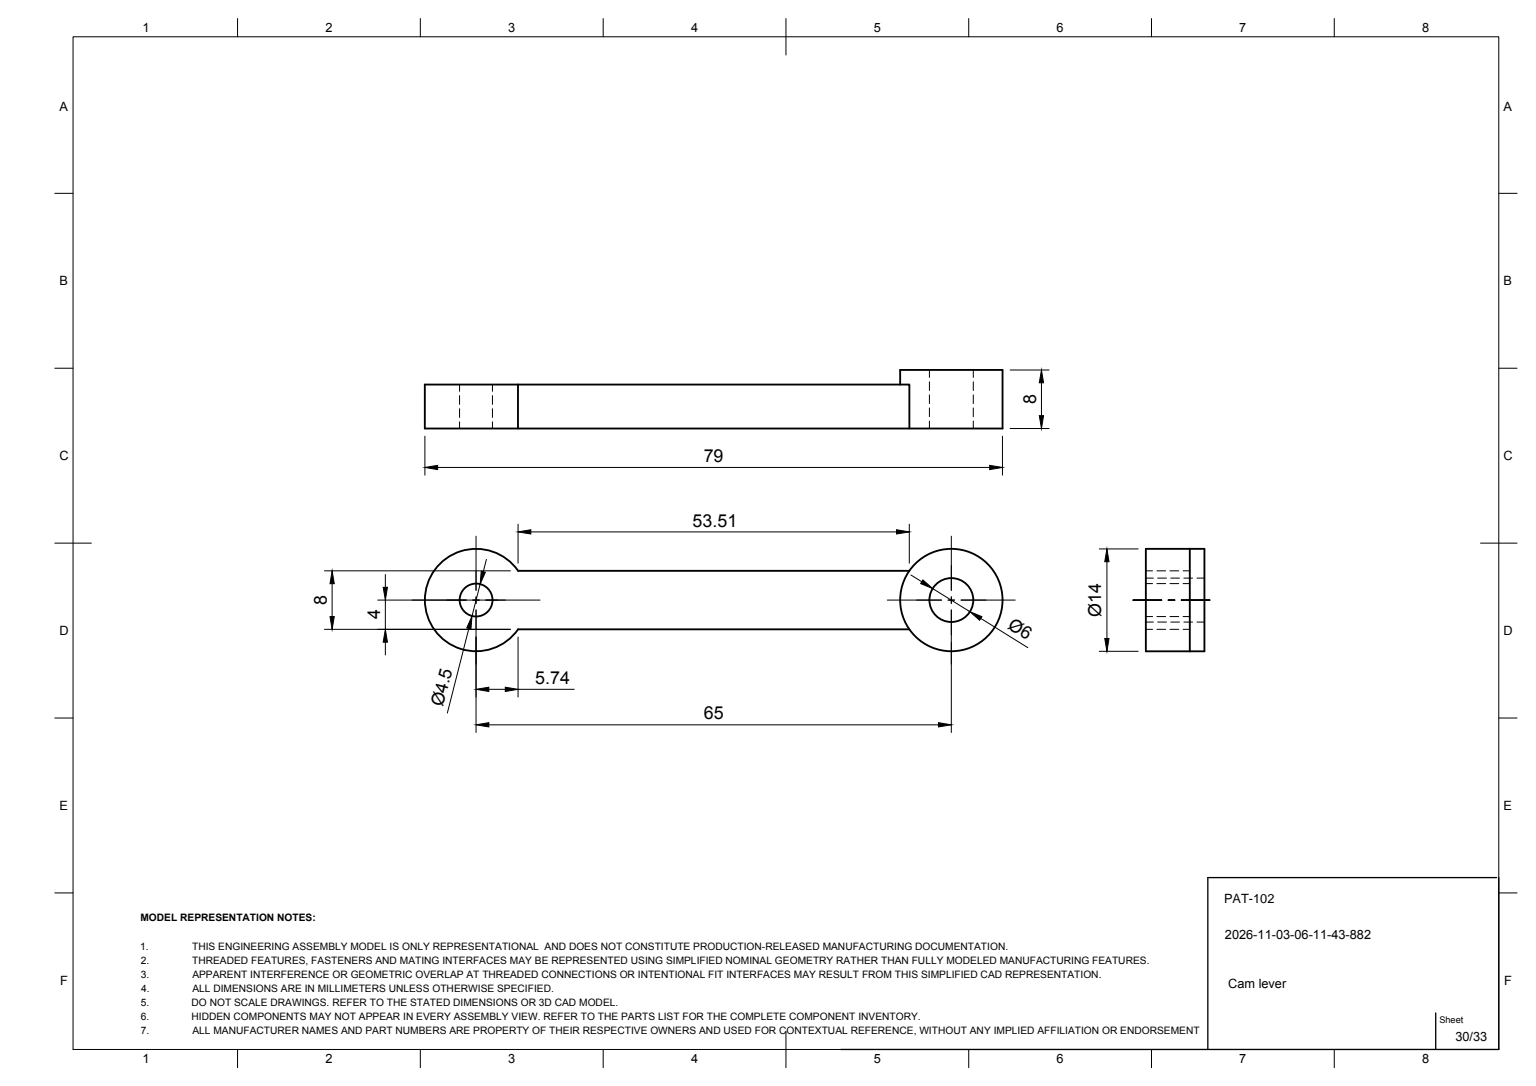
ISO-10303-21;
HEADER;
/* Generated by software containing ST-Developer
 * from STEP Tools, Inc. (www.steptools.com) 
 */

FILE_DESCRIPTION(
/* description */ ('Swing-away clamp arm'),
/* implementation_level */ '2;1');

FILE_NAME(
/* name */ 'Cam lever.step',
/* time_stamp */ '2026-10-28T03:26:03-07:00',
/* author */ (''),
/* organization */ (''),
/* preprocessor_version */ 'ST-DEVELOPER v20.2',
/* originating_system */ 'Autodesk Translation Framework v15.17.0.0',
/* authorisation */ '');

FILE_SCHEMA (('AUTOMOTIVE_DESIGN { 1 0 10303 214 3 1 1 }'));
ENDSEC;

DATA;
#10=MECHANICAL_DESIGN_GEOMETRIC_PRESENTATION_REPRESENTATION('',(#321),#10627);
#261=SHAPE_REPRESENTATION_RELATIONSHIP('SRR','None',#10762,#287);
#287=ADVANCED_BREP_SHAPE_REPRESENTATION('',(#354),#10621);
#321=STYLED_ITEM('',(#10958),#354);
#354=MANIFOLD_SOLID_BREP('Body1',#4928);
#447=FACE_BOUND('',#1288,.T.);
#448=FACE_BOUND('',#1289,.T.);
#449=FACE_BOUND('',#1293,.T.);
#450=FACE_BOUND('',#1297,.T.);
#603=PLANE('',#5751);
#604=PLANE('',#5755);
#605=PLANE('',#5756);
#606=PLANE('',#5757);
#607=PLANE('',#5763);
#889=FACE_OUTER_BOUND('',#1285,.T.);
#890=FACE_OUTER_BOUND('',#1286,.T.);
#891=FACE_OUTER_BOUND('',#1287,.T.);
#892=FACE_OUTER_BOUND('',#1290,.T.);
#893=FACE_OUTER_BOUND('',#1291,.T.);
#894=FACE_OUTER_BOUND('',#1292,.T.);
#895=FACE_OUTER_BOUND('',#1294,.T.);
#896=FACE_OUTER_BOUND('',#1295,.T.);
#897=FACE_OUTER_BOUND('',#1296,.T.);
#1285=EDGE_LOOP('',(#4295,#4296,#4297,#4298));
#1286=EDGE_LOOP('',(#4299,#4300,#4301,#4302));
#1287=EDGE_LOOP('',(#4303,#4304,#4305,#4306,#4307));
#1288=EDGE_LOOP('',(#4308));
#1289=EDGE_LOOP('',(#4309));
#1290=EDGE_LOOP('',(#4310,#4311,#4312,#4313));
#1291=EDGE_LOOP('',(#4314,#4315,#4316,#4317));
#1292=EDGE_LOOP('',(#4318,#4319,#4320,#4321));
#1293=EDGE_LOOP('',(#4322));
#1294=EDGE_LOOP('',(#4323,#4324,#4325,#4326));
#1295=EDGE_LOOP('',(#4327,#4328,#4329,#4330,#4331,#4332,#4333,#4334));
#1296=EDGE_LOOP('',(#4335));
#1297=EDGE_LOOP('',(#4336));
#1609=LINE('',#10314,#1931);
#1610=LINE('',#10319,#1932);
#1611=LINE('',#10323,#1933);
#1612=LINE('',#10327,#1934);
#1613=LINE('',#10332,#1935);
#1614=LINE('',#10337,#1936);
#1615=LINE('',#10338,#1937);
#1616=LINE('',#10341,#1938);
#1617=LINE('',#10342,#1939);
#1618=LINE('',#10348,#1940);
#1619=LINE('',#10352,#1941);
#1931=VECTOR('',#7176,0.225);
#1932=VECTOR('',#7181,1.);
#1933=VECTOR('',#7184,1.);
#1934=VECTOR('',#7189,1.);
#1935=VECTOR('',#7194,1.);
#1936=VECTOR('',#7199,1.);
#1937=VECTOR('',#7200,1.);
#1938=VECTOR('',#7203,1.);
#1939=VECTOR('',#7204,1.);
#1940=VECTOR('',#7213,0.3);
#1941=VECTOR('',#7218,0.7);
#2225=CIRCLE('',#5746,0.225);
#2226=CIRCLE('',#5747,0.225);
#2227=CIRCLE('',#5749,0.699999999999999);
#2228=CIRCLE('',#5750,0.699999999999999);
#2229=CIRCLE('',#5752,0.7);
#2230=CIRCLE('',#5753,0.7);
#2231=CIRCLE('',#5754,0.3);
#2232=CIRCLE('',#5758,0.7);
#2233=CIRCLE('',#5760,0.3);
#2234=CIRCLE('',#5762,0.7);
#2608=VERTEX_POINT('',#10311);
#2609=VERTEX_POINT('',#10313);
#2610=VERTEX_POINT('',#10317);
#2611=VERTEX_POINT('',#10318);
#2612=VERTEX_POINT('',#10320);
#2613=VERTEX_POINT('',#10322);
#2614=VERTEX_POINT('',#10326);
#2615=VERTEX_POINT('',#10328);
#2616=VERTEX_POINT('',#10330);
#2617=VERTEX_POINT('',#10333);
#2618=VERTEX_POINT('',#10336);
#2619=VERTEX_POINT('',#10340);
#2620=VERTEX_POINT('',#10346);
#2621=VERTEX_POINT('',#10350);
#3180=EDGE_CURVE('',#2608,#2608,#2225,.T.);
#3181=EDGE_CURVE('',#2608,#2609,#1609,.T.);
#3182=EDGE_CURVE('',#2609,#2609,#2226,.T.);
#3183=EDGE_CURVE('',#2610,#2611,#1610,.T.);
#3184=EDGE_CURVE('',#2612,#2610,#2227,.T.);
#3185=EDGE_CURVE('',#2613,#2612,#1611,.T.);
#3186=EDGE_CURVE('',#2613,#2611,#2228,.T.);
#3187=EDGE_CURVE('',#2613,#2614,#1612,.T.);
#3188=EDGE_CURVE('',#2615,#2614,#2229,.T.);
#3189=EDGE_CURVE('',#2616,#2615,#2230,.T.);
#3190=EDGE_CURVE('',#2616,#2611,#1613,.T.);
#3191=EDGE_CURVE('',#2617,#2617,#2231,.T.);
#3192=EDGE_CURVE('',#2618,#2612,#1614,.T.);
#3193=EDGE_CURVE('',#2614,#2618,#1615,.T.);
#3194=EDGE_CURVE('',#2619,#2616,#1616,.T.);
#3195=EDGE_CURVE('',#2610,#2619,#1617,.T.);
#3196=EDGE_CURVE('',#2618,#2619,#2232,.T.);
#3197=EDGE_CURVE('',#2620,#2620,#2233,.T.);
#3198=EDGE_CURVE('',#2620,#2617,#1618,.T.);
#3199=EDGE_CURVE('',#2621,#2621,#2234,.T.);
#3200=EDGE_CURVE('',#2621,#2615,#1619,.T.);
#4295=ORIENTED_EDGE('',*,*,#3180,.F.);
#4296=ORIENTED_EDGE('',*,*,#3181,.T.);
#4297=ORIENTED_EDGE('',*,*,#3182,.F.);
#4298=ORIENTED_EDGE('',*,*,#3181,.F.);
#4299=ORIENTED_EDGE('',*,*,#3183,.F.);
#4300=ORIENTED_EDGE('',*,*,#3184,.F.);
#4301=ORIENTED_EDGE('',*,*,#3185,.F.);
#4302=ORIENTED_EDGE('',*,*,#3186,.T.);
#4303=ORIENTED_EDGE('',*,*,#3186,.F.);
#4304=ORIENTED_EDGE('',*,*,#3187,.T.);
#4305=ORIENTED_EDGE('',*,*,#3188,.F.);
#4306=ORIENTED_EDGE('',*,*,#3189,.F.);
#4307=ORIENTED_EDGE('',*,*,#3190,.T.);
#4308=ORIENTED_EDGE('',*,*,#3180,.T.);
#4309=ORIENTED_EDGE('',*,*,#3191,.F.);
#4310=ORIENTED_EDGE('',*,*,#3185,.T.);
#4311=ORIENTED_EDGE('',*,*,#3192,.F.);
#4312=ORIENTED_EDGE('',*,*,#3193,.F.);
#4313=ORIENTED_EDGE('',*,*,#3187,.F.);
#4314=ORIENTED_EDGE('',*,*,#3183,.T.);
#4315=ORIENTED_EDGE('',*,*,#3190,.F.);
#4316=ORIENTED_EDGE('',*,*,#3194,.F.);
#4317=ORIENTED_EDGE('',*,*,#3195,.F.);
#4318=ORIENTED_EDGE('',*,*,#3195,.T.);
#4319=ORIENTED_EDGE('',*,*,#3196,.F.);
#4320=ORIENTED_EDGE('',*,*,#3192,.T.);
#4321=ORIENTED_EDGE('',*,*,#3184,.T.);
#4322=ORIENTED_EDGE('',*,*,#3182,.T.);
#4323=ORIENTED_EDGE('',*,*,#3197,.F.);
#4324=ORIENTED_EDGE('',*,*,#3198,.T.);
#4325=ORIENTED_EDGE('',*,*,#3191,.T.);
#4326=ORIENTED_EDGE('',*,*,#3198,.F.);
#4327=ORIENTED_EDGE('',*,*,#3199,.F.);
#4328=ORIENTED_EDGE('',*,*,#3200,.T.);
#4329=ORIENTED_EDGE('',*,*,#3188,.T.);
#4330=ORIENTED_EDGE('',*,*,#3193,.T.);
#4331=ORIENTED_EDGE('',*,*,#3196,.T.);
#4332=ORIENTED_EDGE('',*,*,#3194,.T.);
#4333=ORIENTED_EDGE('',*,*,#3189,.T.);
#4334=ORIENTED_EDGE('',*,*,#3200,.F.);
#4335=ORIENTED_EDGE('',*,*,#3199,.T.);
#4336=ORIENTED_EDGE('',*,*,#3197,.T.);
#4578=CYLINDRICAL_SURFACE('',#5745,0.225);
#4579=CYLINDRICAL_SURFACE('',#5748,0.699999999999999);
#4580=CYLINDRICAL_SURFACE('',#5759,0.3);
#4581=CYLINDRICAL_SURFACE('',#5761,0.7);
#4844=ADVANCED_FACE('',(#889),#4578,.F.);
#4845=ADVANCED_FACE('',(#890),#4579,.T.);
#4846=ADVANCED_FACE('',(#891,#447,#448),#603,.F.);
#4847=ADVANCED_FACE('',(#892),#604,.T.);
#4848=ADVANCED_FACE('',(#893),#605,.T.);
#4849=ADVANCED_FACE('',(#894,#449),#606,.T.);
#4850=ADVANCED_FACE('',(#895),#4580,.F.);
#4851=ADVANCED_FACE('',(#896),#4581,.T.);
#4852=ADVANCED_FACE('',(#897,#450),#607,.T.);
#4928=CLOSED_SHELL('',(#4844,#4845,#4846,#4847,#4848,#4849,#4850,#4851,
#4852));
#5744=AXIS2_PLACEMENT_3D('',#10309,#7170,#7171);
#5745=AXIS2_PLACEMENT_3D('',#10310,#7172,#7173);
#5746=AXIS2_PLACEMENT_3D('',#10312,#7174,#7175);
#5747=AXIS2_PLACEMENT_3D('',#10315,#7177,#7178);
#5748=AXIS2_PLACEMENT_3D('',#10316,#7179,#7180);
#5749=AXIS2_PLACEMENT_3D('',#10321,#7182,#7183);
#5750=AXIS2_PLACEMENT_3D('',#10324,#7185,#7186);
#5751=AXIS2_PLACEMENT_3D('',#10325,#7187,#7188);
#5752=AXIS2_PLACEMENT_3D('',#10329,#7190,#7191);
#5753=AXIS2_PLACEMENT_3D('',#10331,#7192,#7193);
#5754=AXIS2_PLACEMENT_3D('',#10334,#7195,#7196);
#5755=AXIS2_PLACEMENT_3D('',#10335,#7197,#7198);
#5756=AXIS2_PLACEMENT_3D('',#10339,#7201,#7202);
#5757=AXIS2_PLACEMENT_3D('',#10343,#7205,#7206);
#5758=AXIS2_PLACEMENT_3D('',#10344,#7207,#7208);
#5759=AXIS2_PLACEMENT_3D('',#10345,#7209,#7210);
#5760=AXIS2_PLACEMENT_3D('',#10347,#7211,#7212);
#5761=AXIS2_PLACEMENT_3D('',#10349,#7214,#7215);
#5762=AXIS2_PLACEMENT_3D('',#10351,#7216,#7217);
#5763=AXIS2_PLACEMENT_3D('',#10353,#7219,#7220);
#7170=DIRECTION('axis',(0.,0.,1.));
#7171=DIRECTION('refdir',(1.,0.,0.));
#7172=DIRECTION('center_axis',(0.,1.,0.));
#7173=DIRECTION('ref_axis',(1.,0.,0.));
#7174=DIRECTION('center_axis',(0.,1.,0.));
#7175=DIRECTION('ref_axis',(1.,0.,0.));
#7176=DIRECTION('',(0.,1.,0.));
#7177=DIRECTION('center_axis',(0.,-1.,0.));
#7178=DIRECTION('ref_axis',(1.,0.,0.));
#7179=DIRECTION('center_axis',(0.,1.,0.));
#7180=DIRECTION('ref_axis',(1.,0.,0.));
#7181=DIRECTION('',(0.,-1.,0.));
#7182=DIRECTION('center_axis',(0.,1.,0.));
#7183=DIRECTION('ref_axis',(1.,0.,0.));
#7184=DIRECTION('',(0.,1.,0.));
#7185=DIRECTION('center_axis',(0.,1.,0.));
#7186=DIRECTION('ref_axis',(1.,0.,0.));
#7187=DIRECTION('center_axis',(0.,1.,0.));
#7188=DIRECTION('ref_axis',(1.,0.,0.));
#7189=DIRECTION('',(-1.,0.,0.));
#7190=DIRECTION('center_axis',(0.,1.,0.));
#7191=DIRECTION('ref_axis',(1.,0.,0.));
#7192=DIRECTION('center_axis',(0.,1.,0.));
#7193=DIRECTION('ref_axis',(1.,0.,0.));
#7194=DIRECTION('',(1.,0.,0.));
#7195=DIRECTION('center_axis',(0.,-1.,0.));
#7196=DIRECTION('ref_axis',(1.,0.,0.));
#7197=DIRECTION('center_axis',(0.,0.,1.));
#7198=DIRECTION('ref_axis',(1.,0.,0.));
#7199=DIRECTION('',(1.,0.,0.));
#7200=DIRECTION('',(0.,1.,0.));
#7201=DIRECTION('center_axis',(0.,0.,-1.));
#7202=DIRECTION('ref_axis',(-1.,0.,0.));
#7203=DIRECTION('',(0.,-1.,0.));
#7204=DIRECTION('',(-1.,0.,0.));
#7205=DIRECTION('center_axis',(0.,1.,0.));
#7206=DIRECTION('ref_axis',(0.,0.,1.));
#7207=DIRECTION('center_axis',(0.,1.,0.));
#7208=DIRECTION('ref_axis',(1.,0.,0.));
#7209=DIRECTION('center_axis',(0.,1.,0.));
#7210=DIRECTION('ref_axis',(1.,0.,0.));
#7211=DIRECTION('center_axis',(0.,-1.,0.));
#7212=DIRECTION('ref_axis',(1.,0.,0.));
#7213=DIRECTION('',(0.,-1.,0.));
#7214=DIRECTION('center_axis',(0.,1.,0.));
#7215=DIRECTION('ref_axis',(1.,0.,0.));
#7216=DIRECTION('center_axis',(0.,1.,0.));
#7217=DIRECTION('ref_axis',(1.,0.,0.));
#7218=DIRECTION('',(0.,-1.,0.));
#7219=DIRECTION('center_axis',(0.,1.,0.));
#7220=DIRECTION('ref_axis',(1.,0.,0.));
#10309=CARTESIAN_POINT('',(0.,0.,0.));
#10310=CARTESIAN_POINT('Origin',(8.5,-2.3,10.5));
#10311=CARTESIAN_POINT('',(8.275,-2.2,10.5));
#10312=CARTESIAN_POINT('Origin',(8.5,-2.2,10.5));
#10313=CARTESIAN_POINT('',(8.275,-1.6,10.5));
#10314=CARTESIAN_POINT('',(8.275,-2.3,10.5));
#10315=CARTESIAN_POINT('Origin',(8.5,-1.6,10.5));
#10316=CARTESIAN_POINT('Origin',(8.5,-2.2,10.5));
#10317=CARTESIAN_POINT('',(7.9255437353462,-1.6,10.1));
#10318=CARTESIAN_POINT('',(7.9255437353462,-2.2,10.1));
#10319=CARTESIAN_POINT('',(7.9255437353462,-2.2,10.1));
#10320=CARTESIAN_POINT('',(7.9255437353462,-1.6,10.9));
#10321=CARTESIAN_POINT('Origin',(8.5,-1.6,10.5));
#10322=CARTESIAN_POINT('',(7.9255437353462,-2.2,10.9));
#10323=CARTESIAN_POINT('',(7.9255437353462,-2.2,10.9));
#10324=CARTESIAN_POINT('Origin',(8.5,-2.2,10.5));
#10325=CARTESIAN_POINT('Origin',(2.,-2.2,10.5));
#10326=CARTESIAN_POINT('',(2.5744562646538,-2.2,10.9));
#10327=CARTESIAN_POINT('',(8.5,-2.2,10.9));
#10328=CARTESIAN_POINT('',(1.3,-2.2,10.5));
#10329=CARTESIAN_POINT('Origin',(2.,-2.2,10.5));
#10330=CARTESIAN_POINT('',(2.5744562646538,-2.2,10.1));
#10331=CARTESIAN_POINT('Origin',(2.,-2.2,10.5));
#10332=CARTESIAN_POINT('',(2.,-2.2,10.1));
#10333=CARTESIAN_POINT('',(1.7,-2.2,10.5));
#10334=CARTESIAN_POINT('Origin',(2.,-2.2,10.5));
#10335=CARTESIAN_POINT('Origin',(2.,-2.2,10.9));
#10336=CARTESIAN_POINT('',(2.5744562646538,-1.6,10.9));
#10337=CARTESIAN_POINT('',(8.5,-1.6,10.9));
#10338=CARTESIAN_POINT('',(2.5744562646538,-2.2,10.9));
#10339=CARTESIAN_POINT('Origin',(8.5,-2.2,10.1));
#10340=CARTESIAN_POINT('',(2.5744562646538,-1.6,10.1));
#10341=CARTESIAN_POINT('',(2.5744562646538,-2.2,10.1));
#10342=CARTESIAN_POINT('',(2.,-1.6,10.1));
#10343=CARTESIAN_POINT('Origin',(5.25,-1.6,10.5));
#10344=CARTESIAN_POINT('Origin',(2.,-1.6,10.5));
#10345=CARTESIAN_POINT('Origin',(2.,-2.2,10.5));
#10346=CARTESIAN_POINT('',(1.7,-1.4,10.5));
#10347=CARTESIAN_POINT('Origin',(2.,-1.4,10.5));
#10348=CARTESIAN_POINT('',(1.7,-2.2,10.5));
#10349=CARTESIAN_POINT('Origin',(2.,-2.2,10.5));
#10350=CARTESIAN_POINT('',(1.3,-1.4,10.5));
#10351=CARTESIAN_POINT('Origin',(2.,-1.4,10.5));
#10352=CARTESIAN_POINT('',(1.3,-2.2,10.5));
#10353=CARTESIAN_POINT('Origin',(2.,-1.4,10.5));
#10589=UNCERTAINTY_MEASURE_WITH_UNIT(LENGTH_MEASURE(0.001),#10628,
'DISTANCE_ACCURACY_VALUE',
'Maximum model space distance between geometric entities at asserted c
onnectivities');
#10595=UNCERTAINTY_MEASURE_WITH_UNIT(LENGTH_MEASURE(0.001),#10628,
'DISTANCE_ACCURACY_VALUE',
'Maximum model space distance between geometric entities at asserted c
onnectivities');
#10621=(
GEOMETRIC_REPRESENTATION_CONTEXT(3)
GLOBAL_UNCERTAINTY_ASSIGNED_CONTEXT((#10589))
GLOBAL_UNIT_ASSIGNED_CONTEXT((#10628,#10630,#10631))
REPRESENTATION_CONTEXT('','3D')
);
#10627=(
GEOMETRIC_REPRESENTATION_CONTEXT(3)
GLOBAL_UNCERTAINTY_ASSIGNED_CONTEXT((#10595))
GLOBAL_UNIT_ASSIGNED_CONTEXT((#10628,#10630,#10631))
REPRESENTATION_CONTEXT('','3D')
);
#10628=(
LENGTH_UNIT()
NAMED_UNIT(*)
SI_UNIT(.CENTI.,.METRE.)
);
#10630=(
NAMED_UNIT(*)
PLANE_ANGLE_UNIT()
SI_UNIT($,.RADIAN.)
);
#10631=(
NAMED_UNIT(*)
SI_UNIT($,.STERADIAN.)
SOLID_ANGLE_UNIT()
);
#10657=SHAPE_DEFINITION_REPRESENTATION(#10703,#10762);
#10703=PRODUCT_DEFINITION_SHAPE('',$,#10794);
#10762=SHAPE_REPRESENTATION('',(#5744),#10621);
#10768=PRODUCT_DEFINITION_CONTEXT('part definition',#10863,'design');
#10794=PRODUCT_DEFINITION('Cam lever','Cam lever',#10825,#10768);
#10825=PRODUCT_DEFINITION_FORMATION('',$,#10890);
#10863=APPLICATION_CONTEXT(
'Core Data for Automotive Mechanical Design Process');
#10864=PRODUCT_CONTEXT('part definition',#10863,'mechanical');
#10890=PRODUCT('Cam lever','Cam lever','Cam lever',(#10864));
#10952=COLOUR_RGB('Sky Blue',0.24,0.69,0.87);
#10953=FILL_AREA_STYLE_COLOUR('',#10952);
#10954=FILL_AREA_STYLE('',(#10953));
#10955=SURFACE_STYLE_FILL_AREA(#10954);
#10956=SURFACE_SIDE_STYLE('',(#10955));
#10957=SURFACE_STYLE_USAGE(.BOTH.,#10956);
#10958=PRESENTATION_STYLE_ASSIGNMENT((#10957));
ENDSEC;
END-ISO-10303-21;
